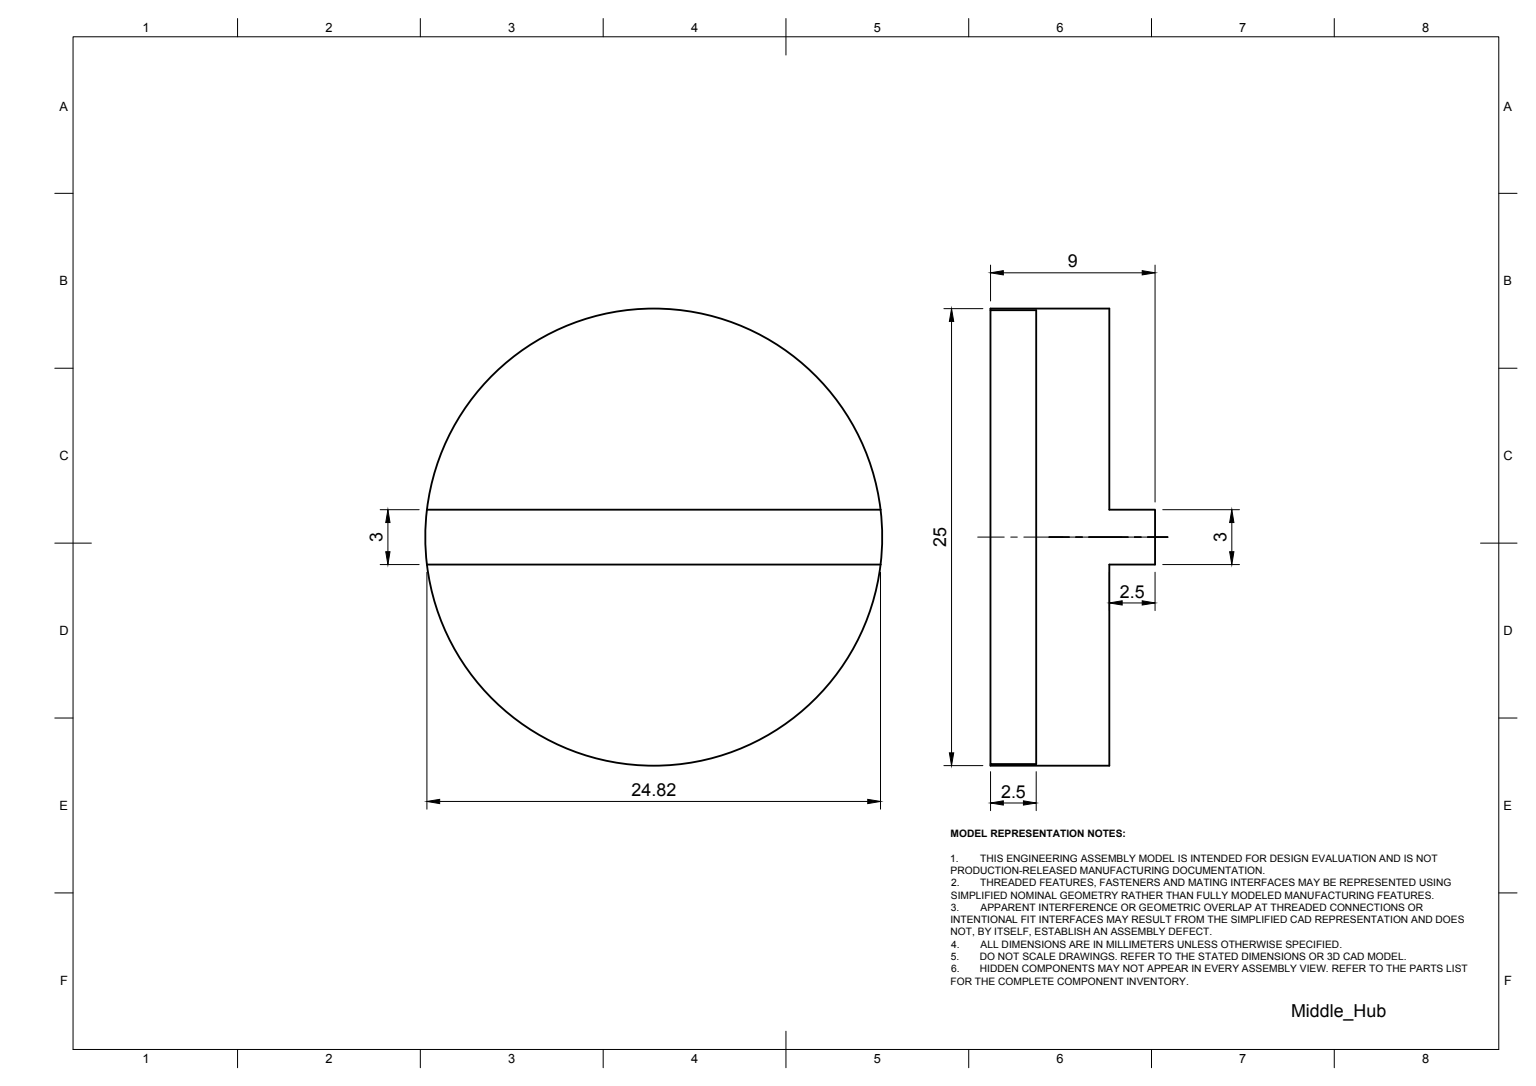
ISO-10303-21;
HEADER;
/* Generated by software containing ST-Developer
 * from STEP Tools, Inc. (www.steptools.com) 
 */

FILE_DESCRIPTION(
/* description */ (''),
/* implementation_level */ '2;1');

FILE_NAME(
/* name */ 'Middle_Hub.step',
/* time_stamp */ '2026-10-05T22:24:12-07:00',
/* author */ (''),
/* organization */ (''),
/* preprocessor_version */ 'ST-DEVELOPER v20.2',
/* originating_system */ 'Autodesk Translation Framework v15.15.0.0',
/* authorisation */ '');

FILE_SCHEMA (('AUTOMOTIVE_DESIGN { 1 0 10303 214 3 1 1 }'));
ENDSEC;

DATA;
#10=MECHANICAL_DESIGN_GEOMETRIC_PRESENTATION_REPRESENTATION('',(#54),#2116);
#40=SHAPE_REPRESENTATION_RELATIONSHIP('SRR','None',#2146,#47);
#47=ADVANCED_BREP_SHAPE_REPRESENTATION('',(#61),#2110);
#54=STYLED_ITEM('',(#2190),#61);
#61=MANIFOLD_SOLID_BREP('Body1',#1148);
#86=PLANE('',#1261);
#87=PLANE('',#1262);
#88=PLANE('',#1263);
#89=PLANE('',#1267);
#90=PLANE('',#1269);
#91=PLANE('',#1271);
#92=PLANE('',#1272);
#93=PLANE('',#1273);
#94=PLANE('',#1276);
#95=PLANE('',#1278);
#146=FACE_OUTER_BOUND('',#217,.T.);
#147=FACE_OUTER_BOUND('',#218,.T.);
#148=FACE_OUTER_BOUND('',#219,.T.);
#149=FACE_OUTER_BOUND('',#220,.T.);
#150=FACE_OUTER_BOUND('',#221,.T.);
#151=FACE_OUTER_BOUND('',#222,.T.);
#152=FACE_OUTER_BOUND('',#223,.T.);
#153=FACE_OUTER_BOUND('',#224,.T.);
#154=FACE_OUTER_BOUND('',#225,.T.);
#155=FACE_OUTER_BOUND('',#226,.T.);
#156=FACE_OUTER_BOUND('',#227,.T.);
#217=EDGE_LOOP('',(#839,#840,#841,#842));
#218=EDGE_LOOP('',(#843,#844,#845,#846));
#219=EDGE_LOOP('',(#847,#848,#849,#850,#851));
#220=EDGE_LOOP('',(#852,#853));
#221=EDGE_LOOP('',(#854,#855));
#222=EDGE_LOOP('',(#856,#857,#858,#859));
#223=EDGE_LOOP('',(#860,#861,#862,#863));
#224=EDGE_LOOP('',(#864,#865,#866,#867));
#225=EDGE_LOOP('',(#868,#869));
#226=EDGE_LOOP('',(#870,#871,#872));
#227=EDGE_LOOP('',(#873,#874,#875,#876,#877,#878,#879,#880,#881,#882,#883,
#884,#885,#886,#887,#888,#889,#890,#891,#892));
#297=LINE('',#1812,#402);
#298=LINE('',#1814,#403);
#299=LINE('',#1816,#404);
#300=LINE('',#1817,#405);
#301=LINE('',#1821,#406);
#302=LINE('',#1823,#407);
#303=LINE('',#1825,#408);
#304=LINE('',#1826,#409);
#305=LINE('',#1839,#410);
#306=LINE('',#1841,#411);
#307=LINE('',#1843,#412);
#308=LINE('',#1844,#413);
#309=LINE('',#1848,#414);
#310=LINE('',#1850,#415);
#311=LINE('',#1852,#416);
#312=LINE('',#1853,#417);
#313=LINE('',#1864,#418);
#402=VECTOR('',#1435,10.);
#403=VECTOR('',#1436,10.);
#404=VECTOR('',#1437,10.);
#405=VECTOR('',#1438,10.);
#406=VECTOR('',#1441,10.);
#407=VECTOR('',#1442,10.);
#408=VECTOR('',#1443,10.);
#409=VECTOR('',#1444,10.);
#410=VECTOR('',#1463,10.);
#411=VECTOR('',#1464,10.);
#412=VECTOR('',#1465,10.);
#413=VECTOR('',#1466,10.);
#414=VECTOR('',#1469,10.);
#415=VECTOR('',#1470,10.);
#416=VECTOR('',#1471,10.);
#417=VECTOR('',#1472,10.);
#418=VECTOR('',#1491,12.5);
#497=CIRCLE('',#1264,12.5);
#498=CIRCLE('',#1265,12.5);
#499=CIRCLE('',#1266,12.5);
#500=CIRCLE('',#1268,12.5);
#501=CIRCLE('',#1270,12.5);
#502=CIRCLE('',#1274,12.5);
#503=CIRCLE('',#1275,12.5);
#504=CIRCLE('',#1277,12.5);
#505=CIRCLE('',#1279,12.5);
#506=CIRCLE('',#1280,12.5);
#548=VERTEX_POINT('',#1810);
#549=VERTEX_POINT('',#1811);
#550=VERTEX_POINT('',#1813);
#551=VERTEX_POINT('',#1815);
#552=VERTEX_POINT('',#1819);
#553=VERTEX_POINT('',#1820);
#554=VERTEX_POINT('',#1822);
#555=VERTEX_POINT('',#1824);
#556=VERTEX_POINT('',#1829);
#557=VERTEX_POINT('',#1837);
#558=VERTEX_POINT('',#1838);
#559=VERTEX_POINT('',#1840);
#560=VERTEX_POINT('',#1842);
#561=VERTEX_POINT('',#1846);
#562=VERTEX_POINT('',#1847);
#563=VERTEX_POINT('',#1849);
#564=VERTEX_POINT('',#1851);
#565=VERTEX_POINT('',#1860);
#658=EDGE_CURVE('',#548,#549,#297,.T.);
#659=EDGE_CURVE('',#548,#550,#298,.T.);
#660=EDGE_CURVE('',#551,#550,#299,.T.);
#661=EDGE_CURVE('',#549,#551,#300,.T.);
#662=EDGE_CURVE('',#552,#553,#301,.T.);
#663=EDGE_CURVE('',#552,#554,#302,.T.);
#664=EDGE_CURVE('',#555,#554,#303,.T.);
#665=EDGE_CURVE('',#553,#555,#304,.T.);
#666=EDGE_CURVE('',#550,#555,#497,.T.);
#667=EDGE_CURVE('',#554,#556,#498,.T.);
#668=EDGE_CURVE('',#556,#551,#499,.T.);
#669=EDGE_CURVE('',#549,#548,#500,.T.);
#670=EDGE_CURVE('',#553,#552,#501,.T.);
#671=EDGE_CURVE('',#557,#558,#305,.T.);
#672=EDGE_CURVE('',#557,#559,#306,.T.);
#673=EDGE_CURVE('',#560,#559,#307,.T.);
#674=EDGE_CURVE('',#558,#560,#308,.T.);
#675=EDGE_CURVE('',#561,#562,#309,.T.);
#676=EDGE_CURVE('',#561,#563,#310,.T.);
#677=EDGE_CURVE('',#564,#563,#311,.T.);
#678=EDGE_CURVE('',#562,#564,#312,.T.);
#679=EDGE_CURVE('',#559,#564,#502,.T.);
#680=EDGE_CURVE('',#563,#560,#503,.T.);
#681=EDGE_CURVE('',#557,#558,#504,.T.);
#682=EDGE_CURVE('',#565,#562,#505,.T.);
#683=EDGE_CURVE('',#561,#565,#506,.T.);
#684=EDGE_CURVE('',#556,#565,#313,.T.);
#839=ORIENTED_EDGE('',*,*,#658,.F.);
#840=ORIENTED_EDGE('',*,*,#659,.T.);
#841=ORIENTED_EDGE('',*,*,#660,.F.);
#842=ORIENTED_EDGE('',*,*,#661,.F.);
#843=ORIENTED_EDGE('',*,*,#662,.F.);
#844=ORIENTED_EDGE('',*,*,#663,.T.);
#845=ORIENTED_EDGE('',*,*,#664,.F.);
#846=ORIENTED_EDGE('',*,*,#665,.F.);
#847=ORIENTED_EDGE('',*,*,#666,.T.);
#848=ORIENTED_EDGE('',*,*,#664,.T.);
#849=ORIENTED_EDGE('',*,*,#667,.T.);
#850=ORIENTED_EDGE('',*,*,#668,.T.);
#851=ORIENTED_EDGE('',*,*,#660,.T.);
#852=ORIENTED_EDGE('',*,*,#658,.T.);
#853=ORIENTED_EDGE('',*,*,#669,.T.);
#854=ORIENTED_EDGE('',*,*,#662,.T.);
#855=ORIENTED_EDGE('',*,*,#670,.T.);
#856=ORIENTED_EDGE('',*,*,#671,.F.);
#857=ORIENTED_EDGE('',*,*,#672,.T.);
#858=ORIENTED_EDGE('',*,*,#673,.F.);
#859=ORIENTED_EDGE('',*,*,#674,.F.);
#860=ORIENTED_EDGE('',*,*,#675,.F.);
#861=ORIENTED_EDGE('',*,*,#676,.T.);
#862=ORIENTED_EDGE('',*,*,#677,.F.);
#863=ORIENTED_EDGE('',*,*,#678,.F.);
#864=ORIENTED_EDGE('',*,*,#679,.T.);
#865=ORIENTED_EDGE('',*,*,#677,.T.);
#866=ORIENTED_EDGE('',*,*,#680,.T.);
#867=ORIENTED_EDGE('',*,*,#673,.T.);
#868=ORIENTED_EDGE('',*,*,#671,.T.);
#869=ORIENTED_EDGE('',*,*,#681,.F.);
#870=ORIENTED_EDGE('',*,*,#675,.T.);
#871=ORIENTED_EDGE('',*,*,#682,.F.);
#872=ORIENTED_EDGE('',*,*,#683,.F.);
#873=ORIENTED_EDGE('',*,*,#667,.F.);
#874=ORIENTED_EDGE('',*,*,#663,.F.);
#875=ORIENTED_EDGE('',*,*,#670,.F.);
#876=ORIENTED_EDGE('',*,*,#665,.T.);
#877=ORIENTED_EDGE('',*,*,#666,.F.);
#878=ORIENTED_EDGE('',*,*,#659,.F.);
#879=ORIENTED_EDGE('',*,*,#669,.F.);
#880=ORIENTED_EDGE('',*,*,#661,.T.);
#881=ORIENTED_EDGE('',*,*,#668,.F.);
#882=ORIENTED_EDGE('',*,*,#684,.T.);
#883=ORIENTED_EDGE('',*,*,#682,.T.);
#884=ORIENTED_EDGE('',*,*,#678,.T.);
#885=ORIENTED_EDGE('',*,*,#679,.F.);
#886=ORIENTED_EDGE('',*,*,#672,.F.);
#887=ORIENTED_EDGE('',*,*,#681,.T.);
#888=ORIENTED_EDGE('',*,*,#674,.T.);
#889=ORIENTED_EDGE('',*,*,#680,.F.);
#890=ORIENTED_EDGE('',*,*,#676,.F.);
#891=ORIENTED_EDGE('',*,*,#683,.T.);
#892=ORIENTED_EDGE('',*,*,#684,.F.);
#1073=CYLINDRICAL_SURFACE('',#1281,12.5);
#1095=ADVANCED_FACE('',(#146),#86,.T.);
#1096=ADVANCED_FACE('',(#147),#87,.T.);
#1097=ADVANCED_FACE('',(#148),#88,.T.);
#1098=ADVANCED_FACE('',(#149),#89,.T.);
#1099=ADVANCED_FACE('',(#150),#90,.T.);
#1100=ADVANCED_FACE('',(#151),#91,.T.);
#1101=ADVANCED_FACE('',(#152),#92,.T.);
#1102=ADVANCED_FACE('',(#153),#93,.F.);
#1103=ADVANCED_FACE('',(#154),#94,.F.);
#1104=ADVANCED_FACE('',(#155),#95,.F.);
#1105=ADVANCED_FACE('',(#156),#1073,.T.);
#1148=CLOSED_SHELL('',(#1095,#1096,#1097,#1098,#1099,#1100,#1101,#1102,
#1103,#1104,#1105));
#1260=AXIS2_PLACEMENT_3D('',#1808,#1431,#1432);
#1261=AXIS2_PLACEMENT_3D('',#1809,#1433,#1434);
#1262=AXIS2_PLACEMENT_3D('',#1818,#1439,#1440);
#1263=AXIS2_PLACEMENT_3D('',#1827,#1445,#1446);
#1264=AXIS2_PLACEMENT_3D('',#1828,#1447,#1448);
#1265=AXIS2_PLACEMENT_3D('',#1830,#1449,#1450);
#1266=AXIS2_PLACEMENT_3D('',#1831,#1451,#1452);
#1267=AXIS2_PLACEMENT_3D('',#1832,#1453,#1454);
#1268=AXIS2_PLACEMENT_3D('',#1833,#1455,#1456);
#1269=AXIS2_PLACEMENT_3D('',#1834,#1457,#1458);
#1270=AXIS2_PLACEMENT_3D('',#1835,#1459,#1460);
#1271=AXIS2_PLACEMENT_3D('',#1836,#1461,#1462);
#1272=AXIS2_PLACEMENT_3D('',#1845,#1467,#1468);
#1273=AXIS2_PLACEMENT_3D('',#1854,#1473,#1474);
#1274=AXIS2_PLACEMENT_3D('',#1855,#1475,#1476);
#1275=AXIS2_PLACEMENT_3D('',#1856,#1477,#1478);
#1276=AXIS2_PLACEMENT_3D('',#1857,#1479,#1480);
#1277=AXIS2_PLACEMENT_3D('',#1858,#1481,#1482);
#1278=AXIS2_PLACEMENT_3D('',#1859,#1483,#1484);
#1279=AXIS2_PLACEMENT_3D('',#1861,#1485,#1486);
#1280=AXIS2_PLACEMENT_3D('',#1862,#1487,#1488);
#1281=AXIS2_PLACEMENT_3D('',#1863,#1489,#1490);
#1431=DIRECTION('axis',(0.,0.,1.));
#1432=DIRECTION('refdir',(1.,0.,0.));
#1433=DIRECTION('center_axis',(0.,0.,-1.));
#1434=DIRECTION('ref_axis',(-1.,0.,0.));
#1435=DIRECTION('',(1.,0.,0.));
#1436=DIRECTION('',(0.,1.,0.));
#1437=DIRECTION('',(-1.,0.,0.));
#1438=DIRECTION('',(0.,1.,0.));
#1439=DIRECTION('center_axis',(0.,0.,1.));
#1440=DIRECTION('ref_axis',(1.,0.,0.));
#1441=DIRECTION('',(-1.,0.,0.));
#1442=DIRECTION('',(0.,1.,0.));
#1443=DIRECTION('',(1.,0.,0.));
#1444=DIRECTION('',(0.,1.,0.));
#1445=DIRECTION('center_axis',(0.,1.,0.));
#1446=DIRECTION('ref_axis',(-1.,0.,0.));
#1447=DIRECTION('center_axis',(0.,1.,0.));
#1448=DIRECTION('ref_axis',(-1.,0.,0.));
#1449=DIRECTION('center_axis',(0.,1.,0.));
#1450=DIRECTION('ref_axis',(-1.,0.,0.));
#1451=DIRECTION('center_axis',(0.,1.,0.));
#1452=DIRECTION('ref_axis',(-1.,0.,0.));
#1453=DIRECTION('center_axis',(0.,1.,0.));
#1454=DIRECTION('ref_axis',(-1.,0.,0.));
#1455=DIRECTION('center_axis',(0.,1.,0.));
#1456=DIRECTION('ref_axis',(-1.,0.,0.));
#1457=DIRECTION('center_axis',(0.,1.,0.));
#1458=DIRECTION('ref_axis',(-1.,0.,0.));
#1459=DIRECTION('center_axis',(0.,1.,0.));
#1460=DIRECTION('ref_axis',(-1.,0.,0.));
#1461=DIRECTION('center_axis',(-1.,0.,0.));
#1462=DIRECTION('ref_axis',(0.,0.,-1.));
#1463=DIRECTION('',(0.,0.,1.));
#1464=DIRECTION('',(0.,-1.,0.));
#1465=DIRECTION('',(0.,0.,-1.));
#1466=DIRECTION('',(0.,-1.,0.));
#1467=DIRECTION('center_axis',(1.,0.,0.));
#1468=DIRECTION('ref_axis',(0.,0.,1.));
#1469=DIRECTION('',(0.,0.,-1.));
#1470=DIRECTION('',(0.,-1.,0.));
#1471=DIRECTION('',(0.,0.,1.));
#1472=DIRECTION('',(0.,-1.,0.));
#1473=DIRECTION('center_axis',(0.,1.,0.));
#1474=DIRECTION('ref_axis',(-1.,0.,0.));
#1475=DIRECTION('center_axis',(0.,-1.,0.));
#1476=DIRECTION('ref_axis',(-1.,0.,0.));
#1477=DIRECTION('center_axis',(0.,-1.,0.));
#1478=DIRECTION('ref_axis',(-1.,0.,0.));
#1479=DIRECTION('center_axis',(0.,1.,0.));
#1480=DIRECTION('ref_axis',(-1.,0.,0.));
#1481=DIRECTION('center_axis',(0.,1.,0.));
#1482=DIRECTION('ref_axis',(-1.,0.,0.));
#1483=DIRECTION('center_axis',(0.,1.,0.));
#1484=DIRECTION('ref_axis',(-1.,0.,0.));
#1485=DIRECTION('center_axis',(0.,1.,0.));
#1486=DIRECTION('ref_axis',(-1.,0.,0.));
#1487=DIRECTION('center_axis',(0.,1.,0.));
#1488=DIRECTION('ref_axis',(-1.,0.,0.));
#1489=DIRECTION('center_axis',(0.,1.,0.));
#1490=DIRECTION('ref_axis',(-1.,0.,0.));
#1491=DIRECTION('',(0.,-1.,0.));
#1808=CARTESIAN_POINT('',(0.,0.,0.));
#1809=CARTESIAN_POINT('Origin',(12.4096736459909,4.,0.499999999999999));
#1810=CARTESIAN_POINT('',(-12.4096736459909,4.,0.499999999999999));
#1811=CARTESIAN_POINT('',(12.4096736459909,4.,0.499999999999999));
#1812=CARTESIAN_POINT('',(6.20483682299543,4.,0.499999999999999));
#1813=CARTESIAN_POINT('',(-12.4096736459909,6.5,0.499999999999999));
#1814=CARTESIAN_POINT('',(-12.4096736459909,4.,0.499999999999999));
#1815=CARTESIAN_POINT('',(12.4096736459909,6.5,0.499999999999999));
#1816=CARTESIAN_POINT('',(-18.9791024697249,6.5,0.499999999999999));
#1817=CARTESIAN_POINT('',(12.4096736459909,4.,0.499999999999999));
#1818=CARTESIAN_POINT('Origin',(-12.4096736459909,4.,3.5));
#1819=CARTESIAN_POINT('',(12.4096736459909,4.,3.5));
#1820=CARTESIAN_POINT('',(-12.4096736459909,4.,3.5));
#1821=CARTESIAN_POINT('',(-6.20483682299543,4.,3.5));
#1822=CARTESIAN_POINT('',(12.4096736459909,6.5,3.5));
#1823=CARTESIAN_POINT('',(12.4096736459909,4.,3.5));
#1824=CARTESIAN_POINT('',(-12.4096736459909,6.5,3.5));
#1825=CARTESIAN_POINT('',(18.9791024697249,6.5,3.5));
#1826=CARTESIAN_POINT('',(-12.4096736459909,4.,3.5));
#1827=CARTESIAN_POINT('Origin',(0.,6.5,2.));
#1828=CARTESIAN_POINT('Origin',(0.,6.5,2.));
#1829=CARTESIAN_POINT('',(12.5,6.5,2.));
#1830=CARTESIAN_POINT('Origin',(0.,6.5,2.));
#1831=CARTESIAN_POINT('Origin',(0.,6.5,2.));
#1832=CARTESIAN_POINT('Origin',(0.,4.,2.));
#1833=CARTESIAN_POINT('Origin',(0.,4.,2.));
#1834=CARTESIAN_POINT('Origin',(0.,4.,2.));
#1835=CARTESIAN_POINT('Origin',(0.,4.,2.));
#1836=CARTESIAN_POINT('Origin',(-1.5,0.,14.4096736459909));
#1837=CARTESIAN_POINT('',(-1.5,0.,-10.4096736459909));
#1838=CARTESIAN_POINT('',(-1.5,0.,14.4096736459909));
#1839=CARTESIAN_POINT('',(-1.5,0.,8.20483682299543));
#1840=CARTESIAN_POINT('',(-1.5,-2.5,-10.4096736459909));
#1841=CARTESIAN_POINT('',(-1.5,0.,-10.4096736459909));
#1842=CARTESIAN_POINT('',(-1.5,-2.5,14.4096736459909));
#1843=CARTESIAN_POINT('',(-1.5,-2.5,17.2595947063511));
#1844=CARTESIAN_POINT('',(-1.5,0.,14.4096736459909));
#1845=CARTESIAN_POINT('Origin',(1.5,0.,-10.4096736459909));
#1846=CARTESIAN_POINT('',(1.5,0.,14.4096736459909));
#1847=CARTESIAN_POINT('',(1.5,0.,-10.4096736459909));
#1848=CARTESIAN_POINT('',(1.5,0.,-4.20483682299543));
#1849=CARTESIAN_POINT('',(1.5,-2.5,14.4096736459909));
#1850=CARTESIAN_POINT('',(1.5,0.,14.4096736459909));
#1851=CARTESIAN_POINT('',(1.5,-2.5,-10.4096736459909));
#1852=CARTESIAN_POINT('',(1.5,-2.5,-13.2595947063511));
#1853=CARTESIAN_POINT('',(1.5,0.,-10.4096736459909));
#1854=CARTESIAN_POINT('Origin',(2.77555756156289E-16,-2.5,2.));
#1855=CARTESIAN_POINT('Origin',(0.,-2.5,2.));
#1856=CARTESIAN_POINT('Origin',(0.,-2.5,2.));
#1857=CARTESIAN_POINT('Origin',(0.,0.,2.));
#1858=CARTESIAN_POINT('Origin',(0.,0.,2.));
#1859=CARTESIAN_POINT('Origin',(0.,0.,2.));
#1860=CARTESIAN_POINT('',(12.5,0.,2.));
#1861=CARTESIAN_POINT('Origin',(0.,0.,2.));
#1862=CARTESIAN_POINT('Origin',(0.,0.,2.));
#1863=CARTESIAN_POINT('Origin',(0.,0.,2.));
#1864=CARTESIAN_POINT('',(12.5,0.,2.));
#2101=UNCERTAINTY_MEASURE_WITH_UNIT(LENGTH_MEASURE(0.01),#2117,
'DISTANCE_ACCURACY_VALUE',
'Maximum model space distance between geometric entities at asserted c
onnectivities');
#2107=UNCERTAINTY_MEASURE_WITH_UNIT(LENGTH_MEASURE(0.01),#2117,
'DISTANCE_ACCURACY_VALUE',
'Maximum model space distance between geometric entities at asserted c
onnectivities');
#2110=(
GEOMETRIC_REPRESENTATION_CONTEXT(3)
GLOBAL_UNCERTAINTY_ASSIGNED_CONTEXT((#2101))
GLOBAL_UNIT_ASSIGNED_CONTEXT((#2117,#2119,#2120))
REPRESENTATION_CONTEXT('','3D')
);
#2116=(
GEOMETRIC_REPRESENTATION_CONTEXT(3)
GLOBAL_UNCERTAINTY_ASSIGNED_CONTEXT((#2107))
GLOBAL_UNIT_ASSIGNED_CONTEXT((#2117,#2119,#2120))
REPRESENTATION_CONTEXT('','3D')
);
#2117=(
LENGTH_UNIT()
NAMED_UNIT(*)
SI_UNIT(.MILLI.,.METRE.)
);
#2119=(
NAMED_UNIT(*)
PLANE_ANGLE_UNIT()
SI_UNIT($,.RADIAN.)
);
#2120=(
NAMED_UNIT(*)
SI_UNIT($,.STERADIAN.)
SOLID_ANGLE_UNIT()
);
#2123=SHAPE_DEFINITION_REPRESENTATION(#2131,#2146);
#2131=PRODUCT_DEFINITION_SHAPE('',$,#2155);
#2146=SHAPE_REPRESENTATION('',(#1260),#2110);
#2152=PRODUCT_DEFINITION_CONTEXT('part definition',#2178,'design');
#2155=PRODUCT_DEFINITION('Middle_Hub','Middle_Hub',#2163,#2152);
#2163=PRODUCT_DEFINITION_FORMATION('',$,#2182);
#2178=APPLICATION_CONTEXT(
'Core Data for Automotive Mechanical Design Process');
#2179=PRODUCT_CONTEXT('part definition',#2178,'mechanical');
#2182=PRODUCT('Middle_Hub','Middle_Hub',$,(#2179));
#2190=PRESENTATION_STYLE_ASSIGNMENT((#2195));
#2195=SURFACE_STYLE_USAGE(.BOTH.,#2200);
#2200=SURFACE_SIDE_STYLE('',(#2205));
#2205=SURFACE_STYLE_FILL_AREA(#2210);
#2210=FILL_AREA_STYLE('Opaque(170,0,255)',(#2215));
#2215=FILL_AREA_STYLE_COLOUR('Opaque(170,0,255)',#2220);
#2220=COLOUR_RGB('Opaque(170,0,255)', 0.66274510, 0.83137255, 0.94901961);
ENDSEC;
END-ISO-10303-21;
